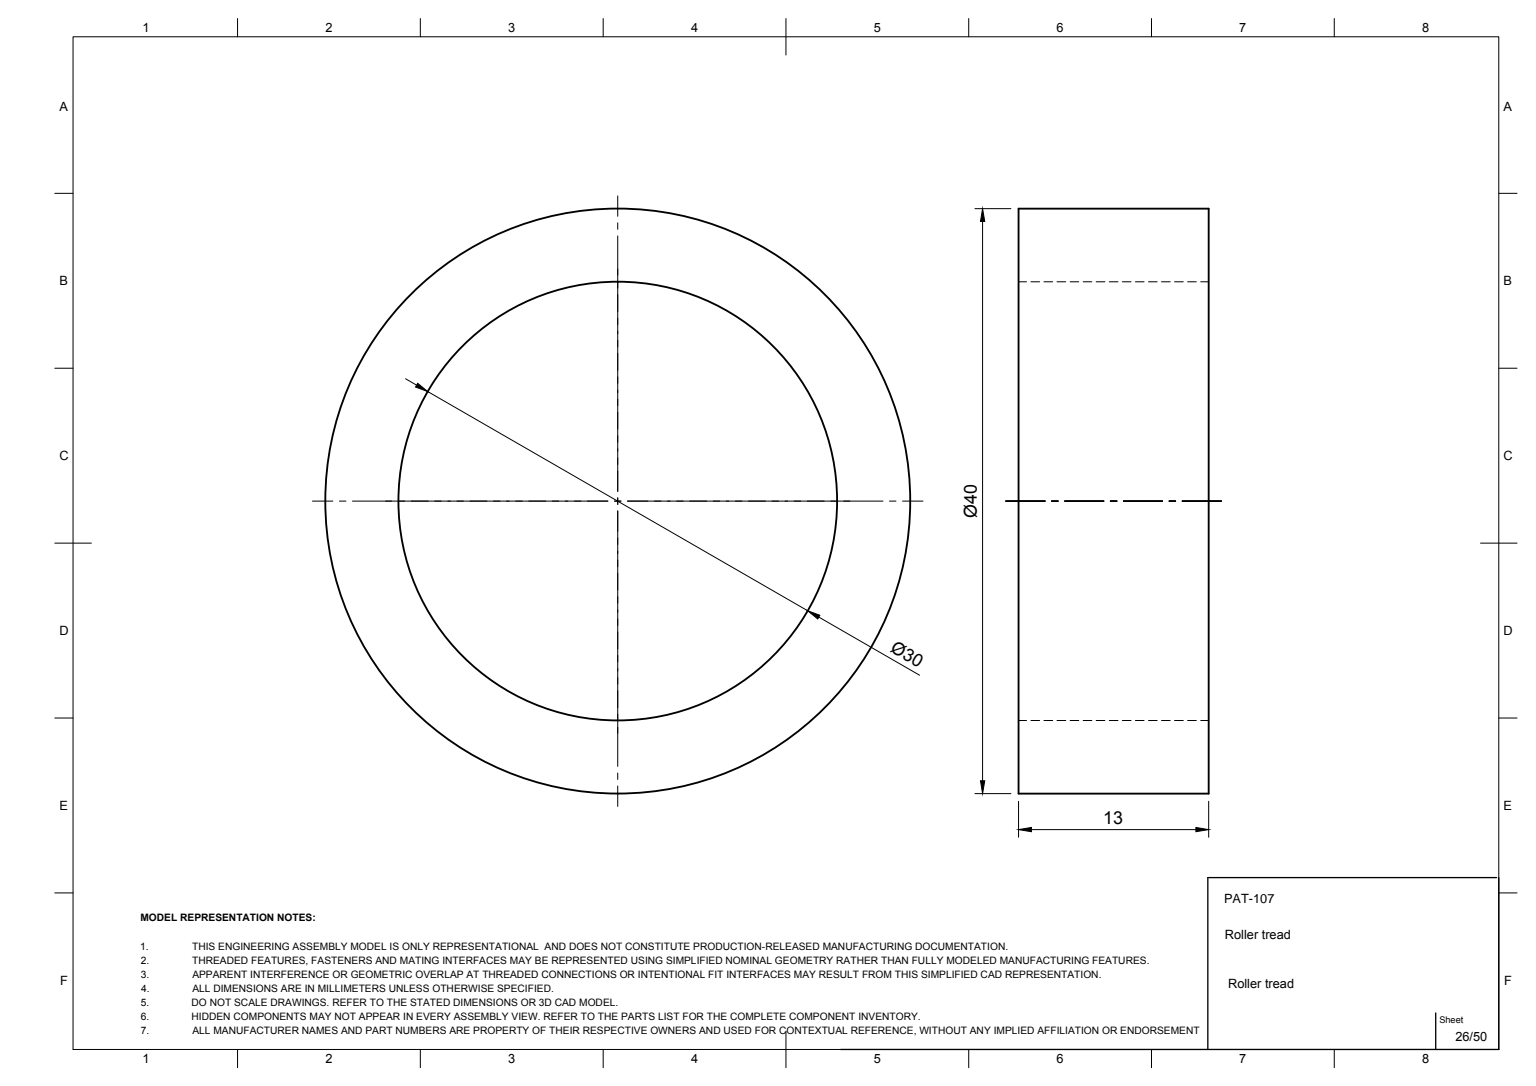
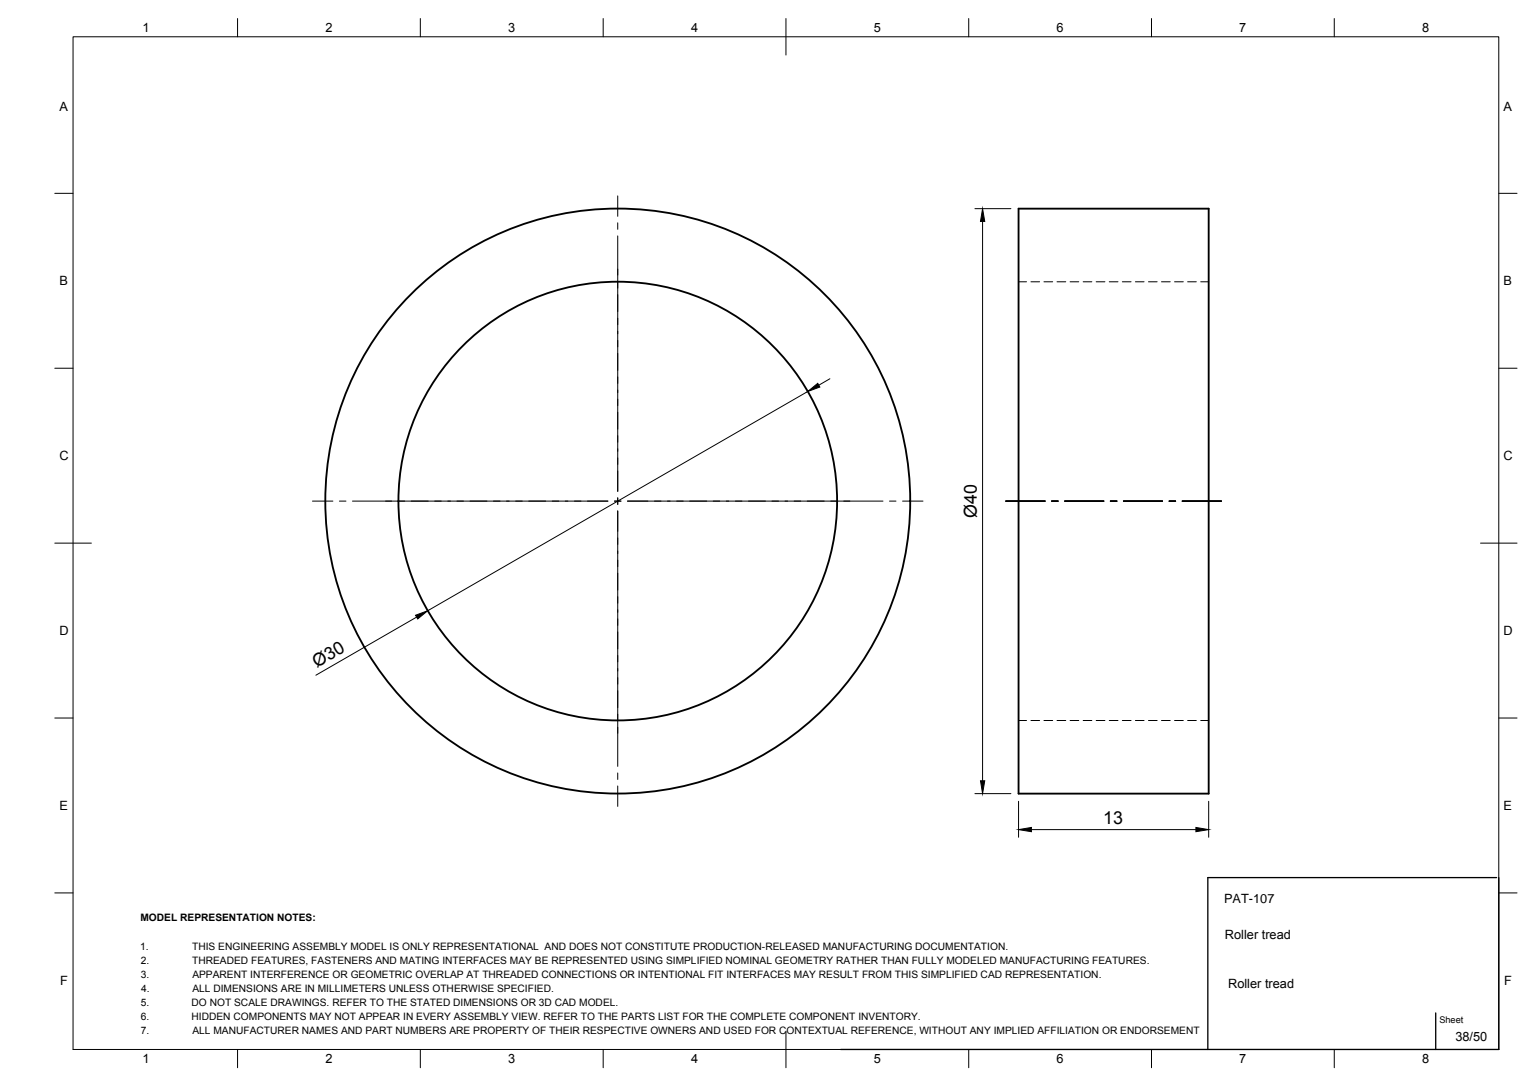
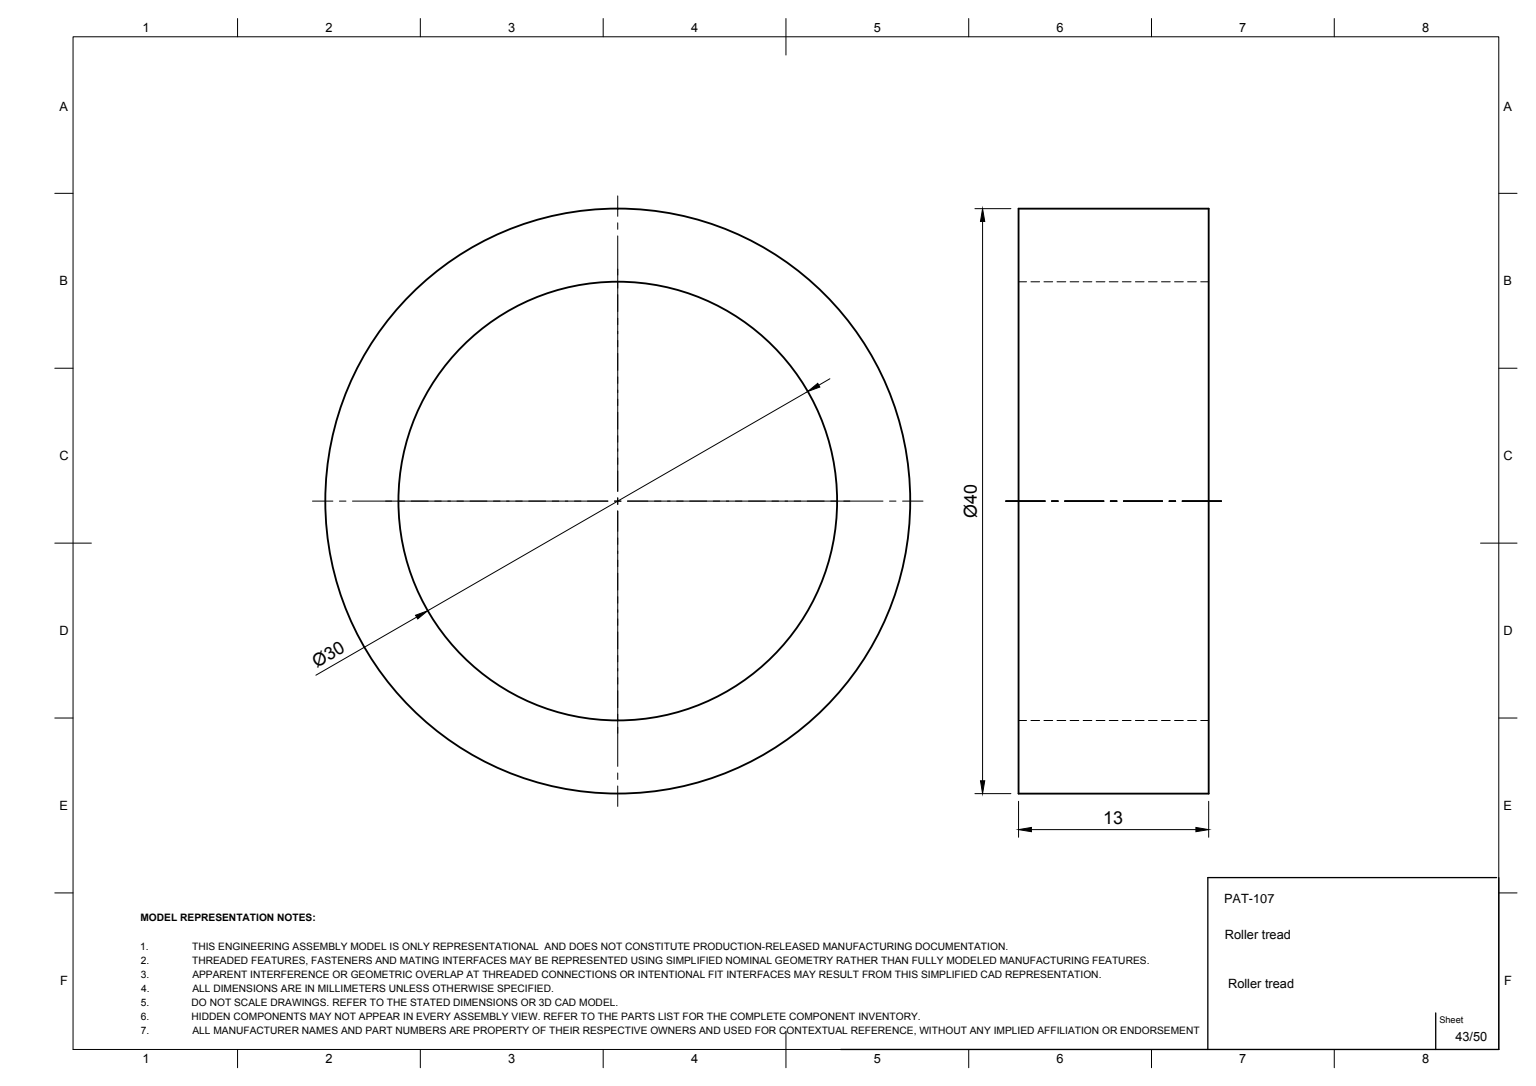
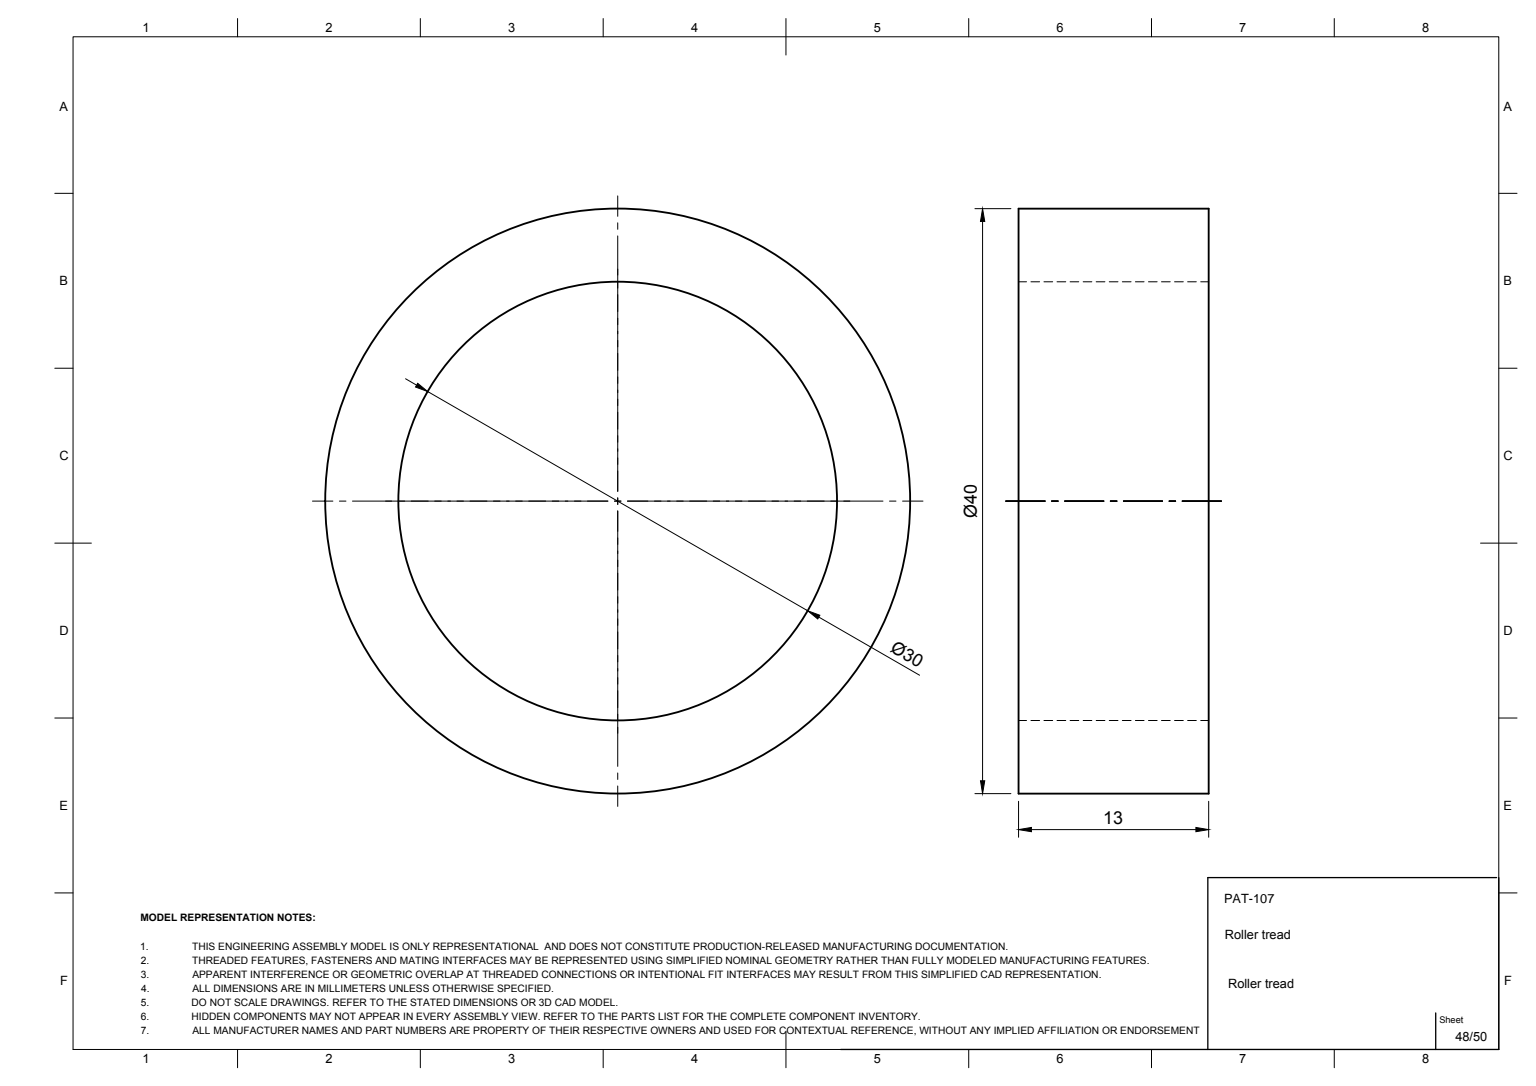
ISO-10303-21;
HEADER;
/* Generated by software containing ST-Developer
 * from STEP Tools, Inc. (www.steptools.com) 
 */

FILE_DESCRIPTION(
/* description */ ('Turntable on roller ring'),
/* implementation_level */ '2;1');

FILE_NAME(
/* name */ 'Roller tread.step',
/* time_stamp */ '2026-10-28T03:23:59-07:00',
/* author */ (''),
/* organization */ (''),
/* preprocessor_version */ 'ST-DEVELOPER v20.2',
/* originating_system */ 'Autodesk Translation Framework v15.17.0.0',
/* authorisation */ '');

FILE_SCHEMA (('AUTOMOTIVE_DESIGN { 1 0 10303 214 3 1 1 }'));
ENDSEC;

DATA;
#10=MECHANICAL_DESIGN_GEOMETRIC_PRESENTATION_REPRESENTATION('',(#664),#16281);
#545=SHAPE_REPRESENTATION_RELATIONSHIP('SRR','None',#16566,#600);
#600=ADVANCED_BREP_SHAPE_REPRESENTATION('',(#732),#16260);
#664=STYLED_ITEM('',(#16925),#732);
#732=MANIFOLD_SOLID_BREP('Body1',#8409);
#957=FACE_BOUND('',#2364,.T.);
#958=FACE_BOUND('',#2366,.T.);
#1209=PLANE('',#9936);
#1210=PLANE('',#9937);
#1656=FACE_OUTER_BOUND('',#2361,.T.);
#1657=FACE_OUTER_BOUND('',#2362,.T.);
#1658=FACE_OUTER_BOUND('',#2363,.T.);
#1659=FACE_OUTER_BOUND('',#2365,.T.);
#2361=EDGE_LOOP('',(#7313,#7314,#7315,#7316));
#2362=EDGE_LOOP('',(#7317,#7318,#7319,#7320));
#2363=EDGE_LOOP('',(#7321));
#2364=EDGE_LOOP('',(#7322));
#2365=EDGE_LOOP('',(#7323));
#2366=EDGE_LOOP('',(#7324));
#2936=LINE('',#15354,#3419);
#2937=LINE('',#15360,#3420);
#3419=VECTOR('',#12427,1.5);
#3420=VECTOR('',#12434,2.);
#3829=CIRCLE('',#9931,1.5);
#3830=CIRCLE('',#9932,1.5);
#3831=CIRCLE('',#9934,2.);
#3832=CIRCLE('',#9935,2.);
#4505=VERTEX_POINT('',#15351);
#4506=VERTEX_POINT('',#15353);
#4507=VERTEX_POINT('',#15357);
#4508=VERTEX_POINT('',#15359);
#5467=EDGE_CURVE('',#4505,#4505,#3829,.T.);
#5468=EDGE_CURVE('',#4505,#4506,#2936,.T.);
#5469=EDGE_CURVE('',#4506,#4506,#3830,.T.);
#5470=EDGE_CURVE('',#4507,#4507,#3831,.T.);
#5471=EDGE_CURVE('',#4507,#4508,#2937,.T.);
#5472=EDGE_CURVE('',#4508,#4508,#3832,.T.);
#7313=ORIENTED_EDGE('',*,*,#5467,.F.);
#7314=ORIENTED_EDGE('',*,*,#5468,.T.);
#7315=ORIENTED_EDGE('',*,*,#5469,.T.);
#7316=ORIENTED_EDGE('',*,*,#5468,.F.);
#7317=ORIENTED_EDGE('',*,*,#5470,.F.);
#7318=ORIENTED_EDGE('',*,*,#5471,.T.);
#7319=ORIENTED_EDGE('',*,*,#5472,.T.);
#7320=ORIENTED_EDGE('',*,*,#5471,.F.);
#7321=ORIENTED_EDGE('',*,*,#5470,.T.);
#7322=ORIENTED_EDGE('',*,*,#5467,.T.);
#7323=ORIENTED_EDGE('',*,*,#5472,.F.);
#7324=ORIENTED_EDGE('',*,*,#5469,.F.);
#7817=CYLINDRICAL_SURFACE('',#9930,1.5);
#7818=CYLINDRICAL_SURFACE('',#9933,2.);
#8259=ADVANCED_FACE('',(#1656),#7817,.F.);
#8260=ADVANCED_FACE('',(#1657),#7818,.T.);
#8261=ADVANCED_FACE('',(#1658,#957),#1209,.T.);
#8262=ADVANCED_FACE('',(#1659,#958),#1210,.F.);
#8409=CLOSED_SHELL('',(#8259,#8260,#8261,#8262));
#9929=AXIS2_PLACEMENT_3D('',#15349,#12421,#12422);
#9930=AXIS2_PLACEMENT_3D('',#15350,#12423,#12424);
#9931=AXIS2_PLACEMENT_3D('',#15352,#12425,#12426);
#9932=AXIS2_PLACEMENT_3D('',#15355,#12428,#12429);
#9933=AXIS2_PLACEMENT_3D('',#15356,#12430,#12431);
#9934=AXIS2_PLACEMENT_3D('',#15358,#12432,#12433);
#9935=AXIS2_PLACEMENT_3D('',#15361,#12435,#12436);
#9936=AXIS2_PLACEMENT_3D('',#15362,#12437,#12438);
#9937=AXIS2_PLACEMENT_3D('',#15363,#12439,#12440);
#12421=DIRECTION('axis',(0.,0.,1.));
#12422=DIRECTION('refdir',(1.,0.,0.));
#12423=DIRECTION('center_axis',(0.,1.,0.));
#12424=DIRECTION('ref_axis',(1.,0.,0.));
#12425=DIRECTION('center_axis',(0.,-1.,0.));
#12426=DIRECTION('ref_axis',(1.,0.,0.));
#12427=DIRECTION('',(0.,-1.,0.));
#12428=DIRECTION('center_axis',(0.,-1.,0.));
#12429=DIRECTION('ref_axis',(1.,0.,0.));
#12430=DIRECTION('center_axis',(0.,1.,0.));
#12431=DIRECTION('ref_axis',(1.,0.,0.));
#12432=DIRECTION('center_axis',(0.,1.,0.));
#12433=DIRECTION('ref_axis',(1.,0.,0.));
#12434=DIRECTION('',(0.,-1.,0.));
#12435=DIRECTION('center_axis',(0.,1.,0.));
#12436=DIRECTION('ref_axis',(1.,0.,0.));
#12437=DIRECTION('center_axis',(0.,1.,0.));
#12438=DIRECTION('ref_axis',(1.,0.,0.));
#12439=DIRECTION('center_axis',(0.,1.,0.));
#12440=DIRECTION('ref_axis',(1.,0.,0.));
#15349=CARTESIAN_POINT('',(0.,0.,0.));
#15350=CARTESIAN_POINT('Origin',(0.,14.35,3.5));
#15351=CARTESIAN_POINT('',(-1.5,15.65,3.5));
#15352=CARTESIAN_POINT('Origin',(0.,15.65,3.5));
#15353=CARTESIAN_POINT('',(-1.5,14.35,3.5));
#15354=CARTESIAN_POINT('',(-1.5,14.35,3.5));
#15355=CARTESIAN_POINT('Origin',(0.,14.35,3.5));
#15356=CARTESIAN_POINT('Origin',(0.,14.35,3.5));
#15357=CARTESIAN_POINT('',(-2.,15.65,3.5));
#15358=CARTESIAN_POINT('Origin',(0.,15.65,3.5));
#15359=CARTESIAN_POINT('',(-2.,14.35,3.5));
#15360=CARTESIAN_POINT('',(-2.,14.35,3.5));
#15361=CARTESIAN_POINT('Origin',(0.,14.35,3.5));
#15362=CARTESIAN_POINT('Origin',(0.,15.65,3.5));
#15363=CARTESIAN_POINT('Origin',(0.,14.35,3.5));
#16191=UNCERTAINTY_MEASURE_WITH_UNIT(LENGTH_MEASURE(0.001),#16282,
'DISTANCE_ACCURACY_VALUE',
'Maximum model space distance between geometric entities at asserted c
onnectivities');
#16212=UNCERTAINTY_MEASURE_WITH_UNIT(LENGTH_MEASURE(0.001),#16282,
'DISTANCE_ACCURACY_VALUE',
'Maximum model space distance between geometric entities at asserted c
onnectivities');
#16260=(
GEOMETRIC_REPRESENTATION_CONTEXT(3)
GLOBAL_UNCERTAINTY_ASSIGNED_CONTEXT((#16191))
GLOBAL_UNIT_ASSIGNED_CONTEXT((#16282,#16284,#16285))
REPRESENTATION_CONTEXT('','3D')
);
#16281=(
GEOMETRIC_REPRESENTATION_CONTEXT(3)
GLOBAL_UNCERTAINTY_ASSIGNED_CONTEXT((#16212))
GLOBAL_UNIT_ASSIGNED_CONTEXT((#16282,#16284,#16285))
REPRESENTATION_CONTEXT('','3D')
);
#16282=(
LENGTH_UNIT()
NAMED_UNIT(*)
SI_UNIT(.CENTI.,.METRE.)
);
#16284=(
NAMED_UNIT(*)
PLANE_ANGLE_UNIT()
SI_UNIT($,.RADIAN.)
);
#16285=(
NAMED_UNIT(*)
SI_UNIT($,.STERADIAN.)
SOLID_ANGLE_UNIT()
);
#16333=SHAPE_DEFINITION_REPRESENTATION(#16467,#16566);
#16467=PRODUCT_DEFINITION_SHAPE('',$,#16635);
#16566=SHAPE_REPRESENTATION('',(#9929),#16260);
#16587=PRODUCT_DEFINITION_CONTEXT('part definition',#16793,'design');
#16635=PRODUCT_DEFINITION('Roller tread','Roller tread',#16703,#16587);
#16703=PRODUCT_DEFINITION_FORMATION('',$,#16842);
#16793=APPLICATION_CONTEXT(
'Core Data for Automotive Mechanical Design Process');
#16794=PRODUCT_CONTEXT('part definition',#16793,'mechanical');
#16842=PRODUCT('Roller tread','Roller tread','Roller tread',(#16794));
#16919=COLOUR_RGB('Sky Blue',0.24,0.69,0.87);
#16920=FILL_AREA_STYLE_COLOUR('',#16919);
#16921=FILL_AREA_STYLE('',(#16920));
#16922=SURFACE_STYLE_FILL_AREA(#16921);
#16923=SURFACE_SIDE_STYLE('',(#16922));
#16924=SURFACE_STYLE_USAGE(.BOTH.,#16923);
#16925=PRESENTATION_STYLE_ASSIGNMENT((#16924));
ENDSEC;
END-ISO-10303-21;
